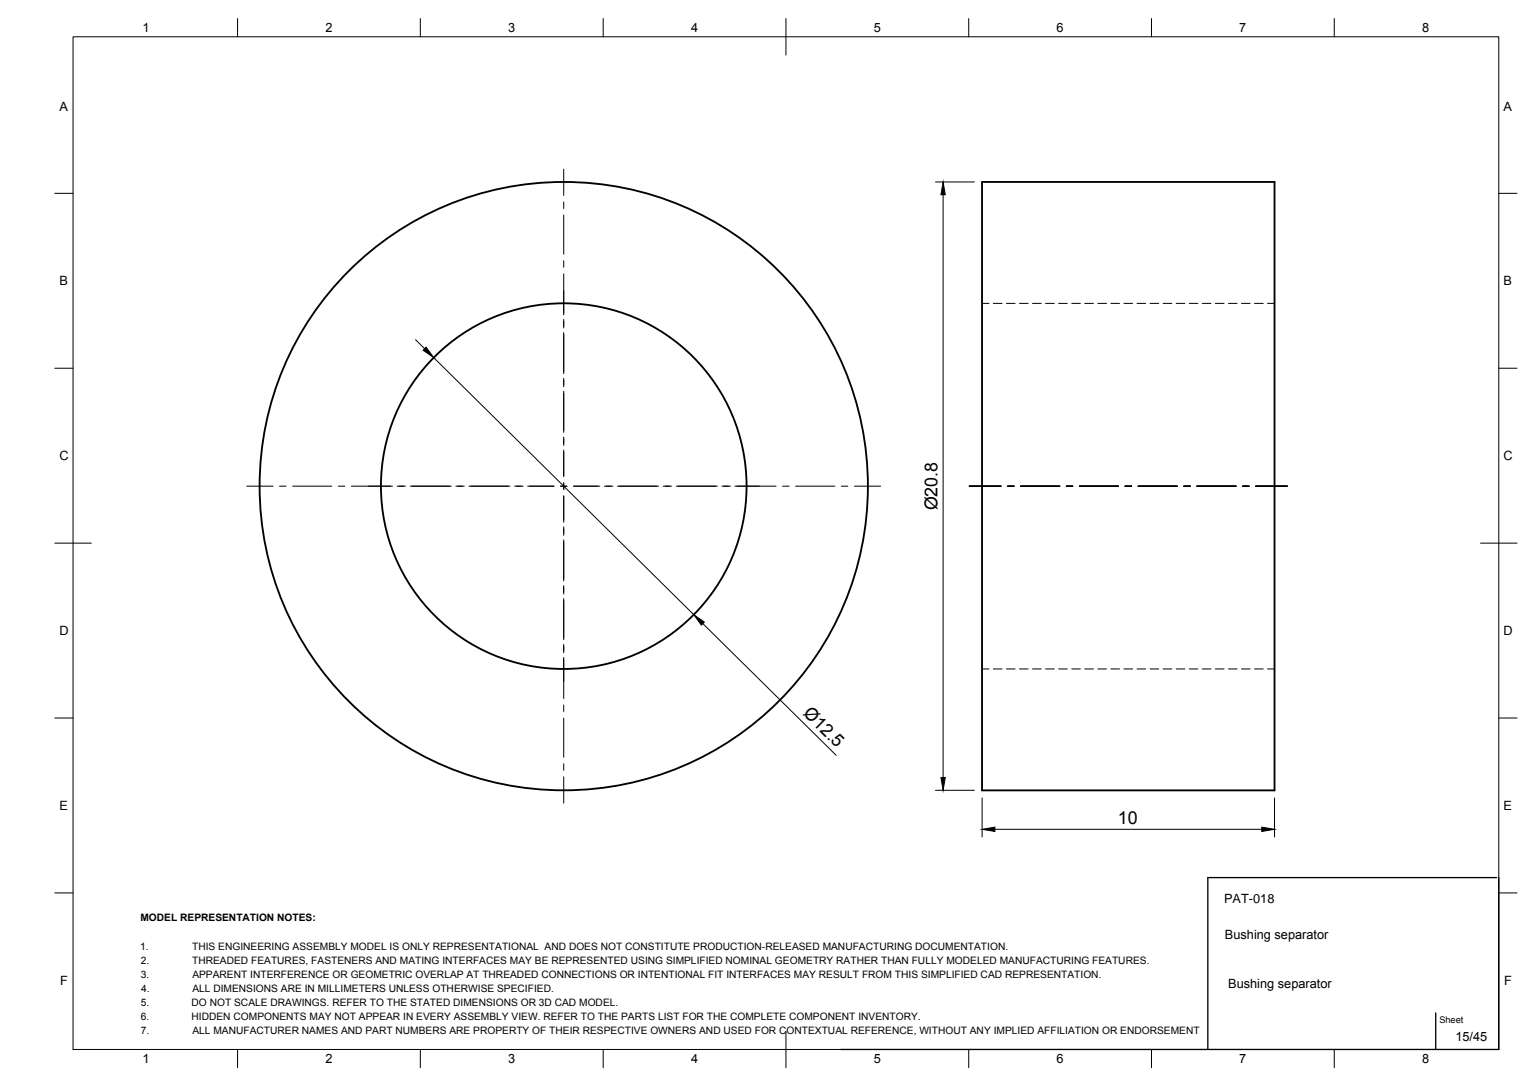
ISO-10303-21;
HEADER;
/* Generated by software containing ST-Developer
 * from STEP Tools, Inc. (www.steptools.com) 
 */

FILE_DESCRIPTION(
/* description */ ('Cam-driven reciprocating slide'),
/* implementation_level */ '2;1');

FILE_NAME(
/* name */ 'Bushing separator.step',
/* time_stamp */ '2026-10-28T03:25:20-07:00',
/* author */ (''),
/* organization */ (''),
/* preprocessor_version */ 'ST-DEVELOPER v20.2',
/* originating_system */ 'Autodesk Translation Framework v15.17.0.0',
/* authorisation */ '');

FILE_SCHEMA (('AUTOMOTIVE_DESIGN { 1 0 10303 214 3 1 1 }'));
ENDSEC;

DATA;
#10=MECHANICAL_DESIGN_GEOMETRIC_PRESENTATION_REPRESENTATION('',(#432),#13277);
#358=SHAPE_REPRESENTATION_RELATIONSHIP('SRR','None',#13451,#395);
#395=ADVANCED_BREP_SHAPE_REPRESENTATION('',(#476),#13246);
#432=STYLED_ITEM('',(#13706),#476);
#476=MANIFOLD_SOLID_BREP('Body1',#6408);
#605=FACE_BOUND('',#1515,.T.);
#606=FACE_BOUND('',#1517,.T.);
#757=PLANE('',#7122);
#758=PLANE('',#7123);
#1035=FACE_OUTER_BOUND('',#1512,.T.);
#1036=FACE_OUTER_BOUND('',#1513,.T.);
#1037=FACE_OUTER_BOUND('',#1514,.T.);
#1038=FACE_OUTER_BOUND('',#1516,.T.);
#1512=EDGE_LOOP('',(#4948,#4949,#4950,#4951));
#1513=EDGE_LOOP('',(#4952,#4953,#4954,#4955));
#1514=EDGE_LOOP('',(#4956));
#1515=EDGE_LOOP('',(#4957));
#1516=EDGE_LOOP('',(#4958));
#1517=EDGE_LOOP('',(#4959));
#2023=LINE('',#10401,#2462);
#2024=LINE('',#10407,#2463);
#2462=VECTOR('',#8389,0.625);
#2463=VECTOR('',#8396,1.04);
#2827=CIRCLE('',#7117,0.625);
#2828=CIRCLE('',#7118,0.625);
#2829=CIRCLE('',#7120,1.04);
#2830=CIRCLE('',#7121,1.04);
#3239=VERTEX_POINT('',#10398);
#3240=VERTEX_POINT('',#10400);
#3241=VERTEX_POINT('',#10404);
#3242=VERTEX_POINT('',#10406);
#3864=EDGE_CURVE('',#3239,#3239,#2827,.T.);
#3865=EDGE_CURVE('',#3239,#3240,#2023,.T.);
#3866=EDGE_CURVE('',#3240,#3240,#2828,.T.);
#3867=EDGE_CURVE('',#3241,#3241,#2829,.T.);
#3868=EDGE_CURVE('',#3241,#3242,#2024,.T.);
#3869=EDGE_CURVE('',#3242,#3242,#2830,.T.);
#4948=ORIENTED_EDGE('',*,*,#3864,.F.);
#4949=ORIENTED_EDGE('',*,*,#3865,.T.);
#4950=ORIENTED_EDGE('',*,*,#3866,.T.);
#4951=ORIENTED_EDGE('',*,*,#3865,.F.);
#4952=ORIENTED_EDGE('',*,*,#3867,.F.);
#4953=ORIENTED_EDGE('',*,*,#3868,.T.);
#4954=ORIENTED_EDGE('',*,*,#3869,.T.);
#4955=ORIENTED_EDGE('',*,*,#3868,.F.);
#4956=ORIENTED_EDGE('',*,*,#3867,.T.);
#4957=ORIENTED_EDGE('',*,*,#3864,.T.);
#4958=ORIENTED_EDGE('',*,*,#3869,.F.);
#4959=ORIENTED_EDGE('',*,*,#3866,.F.);
#5950=CYLINDRICAL_SURFACE('',#7116,0.625);
#5951=CYLINDRICAL_SURFACE('',#7119,1.04);
#6153=ADVANCED_FACE('',(#1035),#5950,.F.);
#6154=ADVANCED_FACE('',(#1036),#5951,.T.);
#6155=ADVANCED_FACE('',(#1037,#605),#757,.T.);
#6156=ADVANCED_FACE('',(#1038,#606),#758,.F.);
#6408=CLOSED_SHELL('',(#6153,#6154,#6155,#6156));
#7115=AXIS2_PLACEMENT_3D('',#10396,#8383,#8384);
#7116=AXIS2_PLACEMENT_3D('',#10397,#8385,#8386);
#7117=AXIS2_PLACEMENT_3D('',#10399,#8387,#8388);
#7118=AXIS2_PLACEMENT_3D('',#10402,#8390,#8391);
#7119=AXIS2_PLACEMENT_3D('',#10403,#8392,#8393);
#7120=AXIS2_PLACEMENT_3D('',#10405,#8394,#8395);
#7121=AXIS2_PLACEMENT_3D('',#10408,#8397,#8398);
#7122=AXIS2_PLACEMENT_3D('',#10409,#8399,#8400);
#7123=AXIS2_PLACEMENT_3D('',#10410,#8401,#8402);
#8383=DIRECTION('axis',(0.,0.,1.));
#8384=DIRECTION('refdir',(1.,0.,0.));
#8385=DIRECTION('center_axis',(0.,0.,1.));
#8386=DIRECTION('ref_axis',(1.,0.,0.));
#8387=DIRECTION('center_axis',(0.,0.,-1.));
#8388=DIRECTION('ref_axis',(1.,0.,0.));
#8389=DIRECTION('',(0.,0.,-1.));
#8390=DIRECTION('center_axis',(0.,0.,-1.));
#8391=DIRECTION('ref_axis',(1.,0.,0.));
#8392=DIRECTION('center_axis',(0.,0.,1.));
#8393=DIRECTION('ref_axis',(1.,0.,0.));
#8394=DIRECTION('center_axis',(0.,0.,1.));
#8395=DIRECTION('ref_axis',(1.,0.,0.));
#8396=DIRECTION('',(0.,0.,-1.));
#8397=DIRECTION('center_axis',(0.,0.,1.));
#8398=DIRECTION('ref_axis',(1.,0.,0.));
#8399=DIRECTION('center_axis',(0.,0.,1.));
#8400=DIRECTION('ref_axis',(1.,0.,0.));
#8401=DIRECTION('center_axis',(0.,0.,1.));
#8402=DIRECTION('ref_axis',(1.,0.,0.));
#10396=CARTESIAN_POINT('',(0.,0.,0.));
#10397=CARTESIAN_POINT('Origin',(0.,0.,15.5));
#10398=CARTESIAN_POINT('',(-0.625,-7.65404249467096E-17,16.5));
#10399=CARTESIAN_POINT('Origin',(0.,0.,16.5));
#10400=CARTESIAN_POINT('',(-0.625,-7.65404249467096E-17,15.5));
#10401=CARTESIAN_POINT('',(-0.625,-7.65404249467096E-17,15.5));
#10402=CARTESIAN_POINT('Origin',(0.,0.,15.5));
#10403=CARTESIAN_POINT('Origin',(0.,0.,15.5));
#10404=CARTESIAN_POINT('',(-1.04,-1.27363267111325E-16,16.5));
#10405=CARTESIAN_POINT('Origin',(0.,0.,16.5));
#10406=CARTESIAN_POINT('',(-1.04,-1.27363267111325E-16,15.5));
#10407=CARTESIAN_POINT('',(-1.04,-1.27363267111325E-16,15.5));
#10408=CARTESIAN_POINT('Origin',(0.,0.,15.5));
#10409=CARTESIAN_POINT('Origin',(0.,0.,16.5));
#10410=CARTESIAN_POINT('Origin',(0.,0.,15.5));
#13202=UNCERTAINTY_MEASURE_WITH_UNIT(LENGTH_MEASURE(0.001),#13278,
'DISTANCE_ACCURACY_VALUE',
'Maximum model space distance between geometric entities at asserted c
onnectivities');
#13233=UNCERTAINTY_MEASURE_WITH_UNIT(LENGTH_MEASURE(0.001),#13278,
'DISTANCE_ACCURACY_VALUE',
'Maximum model space distance between geometric entities at asserted c
onnectivities');
#13246=(
GEOMETRIC_REPRESENTATION_CONTEXT(3)
GLOBAL_UNCERTAINTY_ASSIGNED_CONTEXT((#13202))
GLOBAL_UNIT_ASSIGNED_CONTEXT((#13278,#13280,#13281))
REPRESENTATION_CONTEXT('','3D')
);
#13277=(
GEOMETRIC_REPRESENTATION_CONTEXT(3)
GLOBAL_UNCERTAINTY_ASSIGNED_CONTEXT((#13233))
GLOBAL_UNIT_ASSIGNED_CONTEXT((#13278,#13280,#13281))
REPRESENTATION_CONTEXT('','3D')
);
#13278=(
LENGTH_UNIT()
NAMED_UNIT(*)
SI_UNIT(.CENTI.,.METRE.)
);
#13280=(
NAMED_UNIT(*)
PLANE_ANGLE_UNIT()
SI_UNIT($,.RADIAN.)
);
#13281=(
NAMED_UNIT(*)
SI_UNIT($,.STERADIAN.)
SOLID_ANGLE_UNIT()
);
#13294=SHAPE_DEFINITION_REPRESENTATION(#13337,#13451);
#13337=PRODUCT_DEFINITION_SHAPE('',$,#13495);
#13451=SHAPE_REPRESENTATION('',(#7115),#13246);
#13482=PRODUCT_DEFINITION_CONTEXT('part definition',#13613,'design');
#13495=PRODUCT_DEFINITION('Bushing separator','Bushing separator',#13538,
#13482);
#13538=PRODUCT_DEFINITION_FORMATION('',$,#13627);
#13613=APPLICATION_CONTEXT(
'Core Data for Automotive Mechanical Design Process');
#13614=PRODUCT_CONTEXT('part definition',#13613,'mechanical');
#13627=PRODUCT('Bushing separator','Bushing separator',
'Bushing separator',(#13614));
#13700=COLOUR_RGB('Light Blue',0.38,0.62,0.78);
#13701=FILL_AREA_STYLE_COLOUR('',#13700);
#13702=FILL_AREA_STYLE('',(#13701));
#13703=SURFACE_STYLE_FILL_AREA(#13702);
#13704=SURFACE_SIDE_STYLE('',(#13703));
#13705=SURFACE_STYLE_USAGE(.BOTH.,#13704);
#13706=PRESENTATION_STYLE_ASSIGNMENT((#13705));
ENDSEC;
END-ISO-10303-21;
